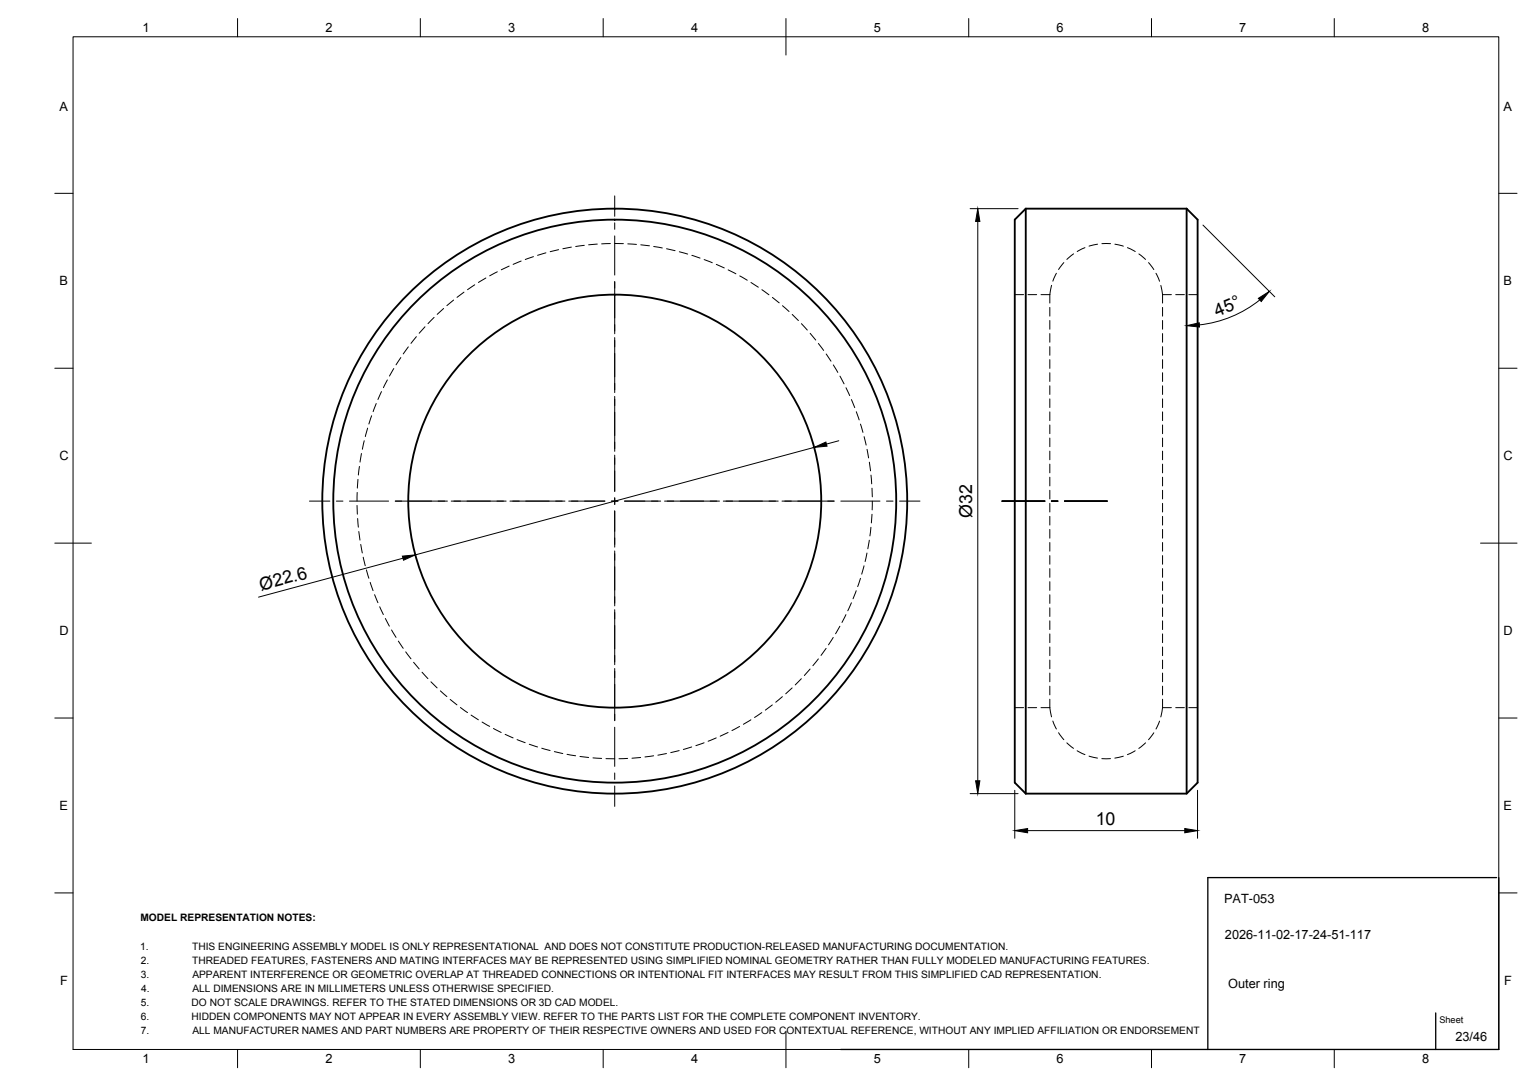
ISO-10303-21;
HEADER;
/* Generated by software containing ST-Developer
 * from STEP Tools, Inc. (www.steptools.com) 
 */

FILE_DESCRIPTION(
/* description */ ('Hand-operated arbor press'),
/* implementation_level */ '2;1');

FILE_NAME(
/* name */ 'Outer ring.step',
/* time_stamp */ '2026-10-28T03:25:25-07:00',
/* author */ (''),
/* organization */ (''),
/* preprocessor_version */ 'ST-DEVELOPER v20.2',
/* originating_system */ 'Autodesk Translation Framework v15.17.0.0',
/* authorisation */ '');

FILE_SCHEMA (('AUTOMOTIVE_DESIGN { 1 0 10303 214 3 1 1 }'));
ENDSEC;

DATA;
#10=MECHANICAL_DESIGN_GEOMETRIC_PRESENTATION_REPRESENTATION('',(#603),#32751);
#472=TOROIDAL_SURFACE('',#13436,1.1,0.309556);
#483=CONICAL_SURFACE('',#13447,1.57,0.785398163397449);
#484=CONICAL_SURFACE('',#13451,1.57,0.785398163397449);
#519=SHAPE_REPRESENTATION_RELATIONSHIP('SRR','None',#32949,#561);
#561=ADVANCED_BREP_SHAPE_REPRESENTATION('',(#651),#32723);
#603=STYLED_ITEM('',(#33242),#651);
#651=MANIFOLD_SOLID_BREP('Body1',#12501);
#804=FACE_BOUND('',#2328,.T.);
#805=FACE_BOUND('',#2333,.T.);
#979=PLANE('',#13444);
#980=PLANE('',#13453);
#1520=FACE_OUTER_BOUND('',#2325,.T.);
#1521=FACE_OUTER_BOUND('',#2326,.T.);
#1522=FACE_OUTER_BOUND('',#2327,.T.);
#1523=FACE_OUTER_BOUND('',#2329,.T.);
#1524=FACE_OUTER_BOUND('',#2330,.T.);
#1525=FACE_OUTER_BOUND('',#2331,.T.);
#1526=FACE_OUTER_BOUND('',#2332,.T.);
#1527=FACE_OUTER_BOUND('',#2334,.T.);
#2325=EDGE_LOOP('',(#9374,#9375,#9376,#9377,#9378,#9379));
#2326=EDGE_LOOP('',(#9380,#9381,#9382,#9383,#9384));
#2327=EDGE_LOOP('',(#9385));
#2328=EDGE_LOOP('',(#9386));
#2329=EDGE_LOOP('',(#9387,#9388,#9389,#9390));
#2330=EDGE_LOOP('',(#9391,#9392,#9393,#9394));
#2331=EDGE_LOOP('',(#9395,#9396,#9397,#9398));
#2332=EDGE_LOOP('',(#9399));
#2333=EDGE_LOOP('',(#9400));
#2334=EDGE_LOOP('',(#9401,#9402,#9403,#9404,#9405));
#3160=LINE('',#18772,#4331);
#3161=LINE('',#18781,#4332);
#3162=LINE('',#18785,#4333);
#3163=LINE('',#18789,#4334);
#3164=LINE('',#18792,#4335);
#4331=VECTOR('',#15381,1.129765);
#4332=VECTOR('',#15392,1.57);
#4333=VECTOR('',#15397,1.6);
#4334=VECTOR('',#15402,1.57);
#4335=VECTOR('',#15407,1.129765);
#5355=CIRCLE('',#13437,1.129765);
#5356=CIRCLE('',#13438,1.129765);
#5357=CIRCLE('',#13439,0.309556);
#5358=CIRCLE('',#13440,1.129765);
#5359=CIRCLE('',#13441,1.129765);
#5360=CIRCLE('',#13443,1.129765);
#5361=CIRCLE('',#13445,1.54);
#5362=CIRCLE('',#13446,1.129765);
#5363=CIRCLE('',#13448,1.6);
#5364=CIRCLE('',#13450,1.6);
#5365=CIRCLE('',#13452,1.54);
#5904=VERTEX_POINT('',#18760);
#5905=VERTEX_POINT('',#18761);
#5906=VERTEX_POINT('',#18764);
#5907=VERTEX_POINT('',#18766);
#5908=VERTEX_POINT('',#18770);
#5909=VERTEX_POINT('',#18774);
#5910=VERTEX_POINT('',#18776);
#5911=VERTEX_POINT('',#18779);
#5912=VERTEX_POINT('',#18783);
#5913=VERTEX_POINT('',#18787);
#7190=EDGE_CURVE('',#5904,#5905,#5355,.T.);
#7191=EDGE_CURVE('',#5905,#5904,#5356,.T.);
#7192=EDGE_CURVE('',#5905,#5906,#5357,.T.);
#7193=EDGE_CURVE('',#5907,#5906,#5358,.T.);
#7194=EDGE_CURVE('',#5906,#5907,#5359,.T.);
#7195=EDGE_CURVE('',#5908,#5908,#5360,.T.);
#7196=EDGE_CURVE('',#5908,#5907,#3160,.T.);
#7197=EDGE_CURVE('',#5909,#5909,#5361,.T.);
#7198=EDGE_CURVE('',#5910,#5910,#5362,.T.);
#7199=EDGE_CURVE('',#5911,#5911,#5363,.T.);
#7200=EDGE_CURVE('',#5911,#5909,#3161,.T.);
#7201=EDGE_CURVE('',#5912,#5912,#5364,.T.);
#7202=EDGE_CURVE('',#5912,#5911,#3162,.T.);
#7203=EDGE_CURVE('',#5913,#5913,#5365,.T.);
#7204=EDGE_CURVE('',#5913,#5912,#3163,.T.);
#7205=EDGE_CURVE('',#5904,#5910,#3164,.T.);
#9374=ORIENTED_EDGE('',*,*,#7190,.F.);
#9375=ORIENTED_EDGE('',*,*,#7191,.F.);
#9376=ORIENTED_EDGE('',*,*,#7192,.T.);
#9377=ORIENTED_EDGE('',*,*,#7193,.F.);
#9378=ORIENTED_EDGE('',*,*,#7194,.F.);
#9379=ORIENTED_EDGE('',*,*,#7192,.F.);
#9380=ORIENTED_EDGE('',*,*,#7195,.T.);
#9381=ORIENTED_EDGE('',*,*,#7196,.T.);
#9382=ORIENTED_EDGE('',*,*,#7193,.T.);
#9383=ORIENTED_EDGE('',*,*,#7194,.T.);
#9384=ORIENTED_EDGE('',*,*,#7196,.F.);
#9385=ORIENTED_EDGE('',*,*,#7197,.F.);
#9386=ORIENTED_EDGE('',*,*,#7198,.T.);
#9387=ORIENTED_EDGE('',*,*,#7199,.F.);
#9388=ORIENTED_EDGE('',*,*,#7200,.T.);
#9389=ORIENTED_EDGE('',*,*,#7197,.T.);
#9390=ORIENTED_EDGE('',*,*,#7200,.F.);
#9391=ORIENTED_EDGE('',*,*,#7201,.F.);
#9392=ORIENTED_EDGE('',*,*,#7202,.T.);
#9393=ORIENTED_EDGE('',*,*,#7199,.T.);
#9394=ORIENTED_EDGE('',*,*,#7202,.F.);
#9395=ORIENTED_EDGE('',*,*,#7203,.F.);
#9396=ORIENTED_EDGE('',*,*,#7204,.T.);
#9397=ORIENTED_EDGE('',*,*,#7201,.T.);
#9398=ORIENTED_EDGE('',*,*,#7204,.F.);
#9399=ORIENTED_EDGE('',*,*,#7203,.T.);
#9400=ORIENTED_EDGE('',*,*,#7195,.F.);
#9401=ORIENTED_EDGE('',*,*,#7190,.T.);
#9402=ORIENTED_EDGE('',*,*,#7191,.T.);
#9403=ORIENTED_EDGE('',*,*,#7205,.T.);
#9404=ORIENTED_EDGE('',*,*,#7198,.F.);
#9405=ORIENTED_EDGE('',*,*,#7205,.F.);
#11732=CYLINDRICAL_SURFACE('',#13442,1.129765);
#11733=CYLINDRICAL_SURFACE('',#13449,1.6);
#11734=CYLINDRICAL_SURFACE('',#13454,1.129765);
#12029=ADVANCED_FACE('',(#1520),#472,.F.);
#12030=ADVANCED_FACE('',(#1521),#11732,.F.);
#12031=ADVANCED_FACE('',(#1522,#804),#979,.T.);
#12032=ADVANCED_FACE('',(#1523),#483,.T.);
#12033=ADVANCED_FACE('',(#1524),#11733,.T.);
#12034=ADVANCED_FACE('',(#1525),#484,.T.);
#12035=ADVANCED_FACE('',(#1526,#805),#980,.T.);
#12036=ADVANCED_FACE('',(#1527),#11734,.F.);
#12501=CLOSED_SHELL('',(#12029,#12030,#12031,#12032,#12033,#12034,#12035,
#12036));
#13435=AXIS2_PLACEMENT_3D('',#18758,#15363,#15364);
#13436=AXIS2_PLACEMENT_3D('',#18759,#15365,#15366);
#13437=AXIS2_PLACEMENT_3D('',#18762,#15367,#15368);
#13438=AXIS2_PLACEMENT_3D('',#18763,#15369,#15370);
#13439=AXIS2_PLACEMENT_3D('',#18765,#15371,#15372);
#13440=AXIS2_PLACEMENT_3D('',#18767,#15373,#15374);
#13441=AXIS2_PLACEMENT_3D('',#18768,#15375,#15376);
#13442=AXIS2_PLACEMENT_3D('',#18769,#15377,#15378);
#13443=AXIS2_PLACEMENT_3D('',#18771,#15379,#15380);
#13444=AXIS2_PLACEMENT_3D('',#18773,#15382,#15383);
#13445=AXIS2_PLACEMENT_3D('',#18775,#15384,#15385);
#13446=AXIS2_PLACEMENT_3D('',#18777,#15386,#15387);
#13447=AXIS2_PLACEMENT_3D('',#18778,#15388,#15389);
#13448=AXIS2_PLACEMENT_3D('',#18780,#15390,#15391);
#13449=AXIS2_PLACEMENT_3D('',#18782,#15393,#15394);
#13450=AXIS2_PLACEMENT_3D('',#18784,#15395,#15396);
#13451=AXIS2_PLACEMENT_3D('',#18786,#15398,#15399);
#13452=AXIS2_PLACEMENT_3D('',#18788,#15400,#15401);
#13453=AXIS2_PLACEMENT_3D('',#18790,#15403,#15404);
#13454=AXIS2_PLACEMENT_3D('',#18791,#15405,#15406);
#15363=DIRECTION('axis',(0.,0.,1.));
#15364=DIRECTION('refdir',(1.,0.,0.));
#15365=DIRECTION('center_axis',(0.,-1.,0.));
#15366=DIRECTION('ref_axis',(0.,0.,-1.));
#15367=DIRECTION('center_axis',(0.,-1.,0.));
#15368=DIRECTION('ref_axis',(1.,0.,0.));
#15369=DIRECTION('center_axis',(0.,-1.,0.));
#15370=DIRECTION('ref_axis',(1.,0.,0.));
#15371=DIRECTION('center_axis',(1.,0.,1.22464679914735E-16));
#15372=DIRECTION('ref_axis',(-1.22464679914735E-16,0.,1.));
#15373=DIRECTION('center_axis',(0.,1.,0.));
#15374=DIRECTION('ref_axis',(1.,0.,0.));
#15375=DIRECTION('center_axis',(0.,1.,0.));
#15376=DIRECTION('ref_axis',(1.,0.,0.));
#15377=DIRECTION('center_axis',(0.,-1.,0.));
#15378=DIRECTION('ref_axis',(1.,0.,0.));
#15379=DIRECTION('center_axis',(0.,-1.,0.));
#15380=DIRECTION('ref_axis',(1.,0.,0.));
#15381=DIRECTION('',(0.,1.,0.));
#15382=DIRECTION('center_axis',(0.,1.,0.));
#15383=DIRECTION('ref_axis',(0.,0.,1.));
#15384=DIRECTION('center_axis',(0.,-1.,0.));
#15385=DIRECTION('ref_axis',(1.,0.,0.));
#15386=DIRECTION('center_axis',(0.,-1.,0.));
#15387=DIRECTION('ref_axis',(1.,0.,0.));
#15388=DIRECTION('center_axis',(0.,-1.,0.));
#15389=DIRECTION('ref_axis',(1.,0.,0.));
#15390=DIRECTION('center_axis',(0.,-1.,0.));
#15391=DIRECTION('ref_axis',(1.,0.,0.));
#15392=DIRECTION('',(0.707106781186548,0.707106781186547,8.65956056235494E-17));
#15393=DIRECTION('center_axis',(0.,-1.,0.));
#15394=DIRECTION('ref_axis',(1.,0.,0.));
#15395=DIRECTION('center_axis',(0.,-1.,0.));
#15396=DIRECTION('ref_axis',(1.,0.,0.));
#15397=DIRECTION('',(0.,1.,0.));
#15398=DIRECTION('center_axis',(0.,1.,0.));
#15399=DIRECTION('ref_axis',(1.,0.,0.));
#15400=DIRECTION('center_axis',(0.,-1.,0.));
#15401=DIRECTION('ref_axis',(1.,0.,0.));
#15402=DIRECTION('',(-0.707106781186548,0.707106781186547,-8.65956056235494E-17));
#15403=DIRECTION('center_axis',(0.,-1.,0.));
#15404=DIRECTION('ref_axis',(0.,0.,-1.));
#15405=DIRECTION('center_axis',(0.,-1.,0.));
#15406=DIRECTION('ref_axis',(1.,0.,0.));
#15407=DIRECTION('',(0.,1.,0.));
#18758=CARTESIAN_POINT('',(0.,0.,0.));
#18759=CARTESIAN_POINT('Origin',(0.,0.,0.));
#18760=CARTESIAN_POINT('',(-1.129765,0.308121667383195,-1.38356309103871E-16));
#18761=CARTESIAN_POINT('',(-1.38356309103871E-16,0.308121667383195,1.129765));
#18762=CARTESIAN_POINT('Origin',(0.,0.308121667383195,0.));
#18763=CARTESIAN_POINT('Origin',(0.,0.308121667383195,0.));
#18764=CARTESIAN_POINT('',(-1.38356309103871E-16,-0.308121667383195,1.129765));
#18765=CARTESIAN_POINT('Origin',(-1.34711147906209E-16,0.,1.1));
#18766=CARTESIAN_POINT('',(-1.129765,-0.308121667383195,1.38356309103871E-16));
#18767=CARTESIAN_POINT('Origin',(0.,-0.308121667383195,0.));
#18768=CARTESIAN_POINT('Origin',(0.,-0.308121667383195,0.));
#18769=CARTESIAN_POINT('Origin',(0.,0.,0.));
#18770=CARTESIAN_POINT('',(-1.129765,-0.5,-1.38356309103871E-16));
#18771=CARTESIAN_POINT('Origin',(0.,-0.5,0.));
#18772=CARTESIAN_POINT('',(-1.129765,0.,-1.38356309103871E-16));
#18773=CARTESIAN_POINT('Origin',(1.54,0.5,0.));
#18774=CARTESIAN_POINT('',(-1.54,0.5,-1.88595607068692E-16));
#18775=CARTESIAN_POINT('Origin',(0.,0.5,0.));
#18776=CARTESIAN_POINT('',(-1.129765,0.5,-1.38356309103871E-16));
#18777=CARTESIAN_POINT('Origin',(0.,0.5,0.));
#18778=CARTESIAN_POINT('Origin',(0.,0.47,0.));
#18779=CARTESIAN_POINT('',(-1.6,0.44,-1.95943487863577E-16));
#18780=CARTESIAN_POINT('Origin',(0.,0.44,0.));
#18781=CARTESIAN_POINT('',(-1.57,0.47,-1.92269547466134E-16));
#18782=CARTESIAN_POINT('Origin',(0.,0.,0.));
#18783=CARTESIAN_POINT('',(-1.6,-0.44,-1.95943487863577E-16));
#18784=CARTESIAN_POINT('Origin',(0.,-0.44,0.));
#18785=CARTESIAN_POINT('',(-1.6,0.,-1.95943487863577E-16));
#18786=CARTESIAN_POINT('Origin',(0.,-0.47,0.));
#18787=CARTESIAN_POINT('',(-1.54,-0.5,-1.88595607068692E-16));
#18788=CARTESIAN_POINT('Origin',(0.,-0.5,0.));
#18789=CARTESIAN_POINT('',(-1.57,-0.47,-1.92269547466134E-16));
#18790=CARTESIAN_POINT('Origin',(1.129765,-0.5,0.));
#18791=CARTESIAN_POINT('Origin',(0.,0.,0.));
#18792=CARTESIAN_POINT('',(-1.129765,0.,-1.38356309103871E-16));
#32674=UNCERTAINTY_MEASURE_WITH_UNIT(LENGTH_MEASURE(0.001),#32752,
'DISTANCE_ACCURACY_VALUE',
'Maximum model space distance between geometric entities at asserted c
onnectivities');
#32702=UNCERTAINTY_MEASURE_WITH_UNIT(LENGTH_MEASURE(0.001),#32752,
'DISTANCE_ACCURACY_VALUE',
'Maximum model space distance between geometric entities at asserted c
onnectivities');
#32723=(
GEOMETRIC_REPRESENTATION_CONTEXT(3)
GLOBAL_UNCERTAINTY_ASSIGNED_CONTEXT((#32674))
GLOBAL_UNIT_ASSIGNED_CONTEXT((#32752,#32754,#32755))
REPRESENTATION_CONTEXT('','3D')
);
#32751=(
GEOMETRIC_REPRESENTATION_CONTEXT(3)
GLOBAL_UNCERTAINTY_ASSIGNED_CONTEXT((#32702))
GLOBAL_UNIT_ASSIGNED_CONTEXT((#32752,#32754,#32755))
REPRESENTATION_CONTEXT('','3D')
);
#32752=(
LENGTH_UNIT()
NAMED_UNIT(*)
SI_UNIT(.CENTI.,.METRE.)
);
#32754=(
NAMED_UNIT(*)
PLANE_ANGLE_UNIT()
SI_UNIT($,.RADIAN.)
);
#32755=(
NAMED_UNIT(*)
SI_UNIT($,.STERADIAN.)
SOLID_ANGLE_UNIT()
);
#32776=SHAPE_DEFINITION_REPRESENTATION(#32824,#32949);
#32824=PRODUCT_DEFINITION_SHAPE('',$,#32998);
#32949=SHAPE_REPRESENTATION('',(#13435),#32723);
#32977=PRODUCT_DEFINITION_CONTEXT('part definition',#33123,'design');
#32998=PRODUCT_DEFINITION('Outer ring','Outer ring',#33046,#32977);
#33046=PRODUCT_DEFINITION_FORMATION('',$,#33145);
#33123=APPLICATION_CONTEXT(
'Core Data for Automotive Mechanical Design Process');
#33124=PRODUCT_CONTEXT('part definition',#33123,'mechanical');
#33145=PRODUCT('Outer ring','Outer ring','Outer ring',(#33124));
#33236=COLOUR_RGB('Grey',0.48,0.52,0.57);
#33237=FILL_AREA_STYLE_COLOUR('',#33236);
#33238=FILL_AREA_STYLE('',(#33237));
#33239=SURFACE_STYLE_FILL_AREA(#33238);
#33240=SURFACE_SIDE_STYLE('',(#33239));
#33241=SURFACE_STYLE_USAGE(.BOTH.,#33240);
#33242=PRESENTATION_STYLE_ASSIGNMENT((#33241));
ENDSEC;
END-ISO-10303-21;
